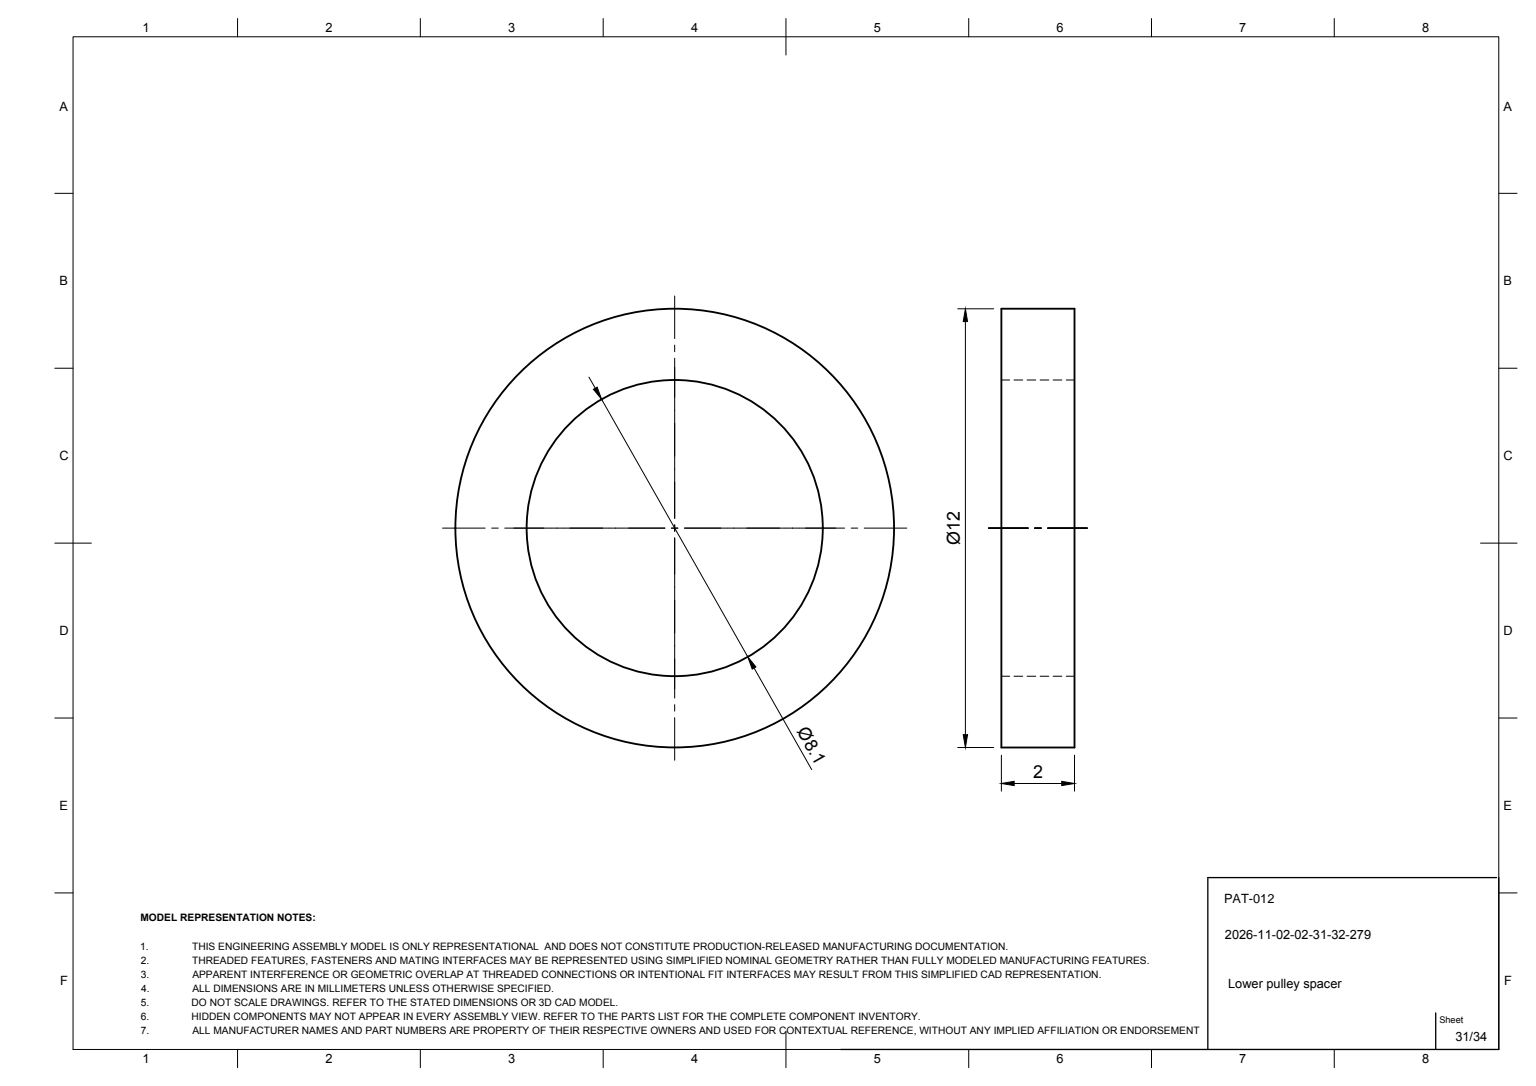
ISO-10303-21;
HEADER;
/* Generated by software containing ST-Developer
 * from STEP Tools, Inc. (www.steptools.com) 
 */

FILE_DESCRIPTION(
/* description */ ('Belt tensioner idler arm'),
/* implementation_level */ '2;1');

FILE_NAME(
/* name */ 'Lower pulley spacer.step',
/* time_stamp */ '2026-10-28T03:22:15-07:00',
/* author */ (''),
/* organization */ (''),
/* preprocessor_version */ 'ST-DEVELOPER v20.2',
/* originating_system */ 'Autodesk Translation Framework v15.17.0.0',
/* authorisation */ '');

FILE_SCHEMA (('AUTOMOTIVE_DESIGN { 1 0 10303 214 3 1 1 }'));
ENDSEC;

DATA;
#10=MECHANICAL_DESIGN_GEOMETRIC_PRESENTATION_REPRESENTATION('',(#481),#12779);
#405=SHAPE_REPRESENTATION_RELATIONSHIP('SRR','None',#12954,#439);
#439=ADVANCED_BREP_SHAPE_REPRESENTATION('',(#520),#12771);
#481=STYLED_ITEM('',(#13177),#520);
#520=MANIFOLD_SOLID_BREP('Body1',#6218);
#644=FACE_BOUND('',#1593,.T.);
#645=FACE_BOUND('',#1595,.T.);
#802=PLANE('',#7188);
#803=PLANE('',#7189);
#1106=FACE_OUTER_BOUND('',#1590,.T.);
#1107=FACE_OUTER_BOUND('',#1591,.T.);
#1108=FACE_OUTER_BOUND('',#1592,.T.);
#1109=FACE_OUTER_BOUND('',#1594,.T.);
#1590=EDGE_LOOP('',(#5188,#5189,#5190,#5191));
#1591=EDGE_LOOP('',(#5192,#5193,#5194,#5195));
#1592=EDGE_LOOP('',(#5196));
#1593=EDGE_LOOP('',(#5197));
#1594=EDGE_LOOP('',(#5198));
#1595=EDGE_LOOP('',(#5199));
#1955=LINE('',#11892,#2304);
#1956=LINE('',#11898,#2305);
#2304=VECTOR('',#8845,0.404999999999999);
#2305=VECTOR('',#8852,0.6);
#2655=CIRCLE('',#7183,0.404999999999999);
#2656=CIRCLE('',#7184,0.404999999999999);
#2657=CIRCLE('',#7186,0.6);
#2658=CIRCLE('',#7187,0.6);
#3138=VERTEX_POINT('',#11889);
#3139=VERTEX_POINT('',#11891);
#3140=VERTEX_POINT('',#11895);
#3141=VERTEX_POINT('',#11897);
#3849=EDGE_CURVE('',#3138,#3138,#2655,.T.);
#3850=EDGE_CURVE('',#3138,#3139,#1955,.T.);
#3851=EDGE_CURVE('',#3139,#3139,#2656,.T.);
#3852=EDGE_CURVE('',#3140,#3140,#2657,.T.);
#3853=EDGE_CURVE('',#3140,#3141,#1956,.T.);
#3854=EDGE_CURVE('',#3141,#3141,#2658,.T.);
#5188=ORIENTED_EDGE('',*,*,#3849,.F.);
#5189=ORIENTED_EDGE('',*,*,#3850,.T.);
#5190=ORIENTED_EDGE('',*,*,#3851,.T.);
#5191=ORIENTED_EDGE('',*,*,#3850,.F.);
#5192=ORIENTED_EDGE('',*,*,#3852,.F.);
#5193=ORIENTED_EDGE('',*,*,#3853,.T.);
#5194=ORIENTED_EDGE('',*,*,#3854,.T.);
#5195=ORIENTED_EDGE('',*,*,#3853,.F.);
#5196=ORIENTED_EDGE('',*,*,#3852,.T.);
#5197=ORIENTED_EDGE('',*,*,#3849,.T.);
#5198=ORIENTED_EDGE('',*,*,#3854,.F.);
#5199=ORIENTED_EDGE('',*,*,#3851,.F.);
#5755=CYLINDRICAL_SURFACE('',#7182,0.404999999999999);
#5756=CYLINDRICAL_SURFACE('',#7185,0.6);
#6083=ADVANCED_FACE('',(#1106),#5755,.F.);
#6084=ADVANCED_FACE('',(#1107),#5756,.T.);
#6085=ADVANCED_FACE('',(#1108,#644),#802,.T.);
#6086=ADVANCED_FACE('',(#1109,#645),#803,.F.);
#6218=CLOSED_SHELL('',(#6083,#6084,#6085,#6086));
#7181=AXIS2_PLACEMENT_3D('',#11887,#8839,#8840);
#7182=AXIS2_PLACEMENT_3D('',#11888,#8841,#8842);
#7183=AXIS2_PLACEMENT_3D('',#11890,#8843,#8844);
#7184=AXIS2_PLACEMENT_3D('',#11893,#8846,#8847);
#7185=AXIS2_PLACEMENT_3D('',#11894,#8848,#8849);
#7186=AXIS2_PLACEMENT_3D('',#11896,#8850,#8851);
#7187=AXIS2_PLACEMENT_3D('',#11899,#8853,#8854);
#7188=AXIS2_PLACEMENT_3D('',#11900,#8855,#8856);
#7189=AXIS2_PLACEMENT_3D('',#11901,#8857,#8858);
#8839=DIRECTION('axis',(0.,0.,1.));
#8840=DIRECTION('refdir',(1.,0.,0.));
#8841=DIRECTION('center_axis',(0.,0.,1.));
#8842=DIRECTION('ref_axis',(1.,0.,0.));
#8843=DIRECTION('center_axis',(0.,0.,-1.));
#8844=DIRECTION('ref_axis',(1.,0.,0.));
#8845=DIRECTION('',(0.,0.,-1.));
#8846=DIRECTION('center_axis',(0.,0.,-1.));
#8847=DIRECTION('ref_axis',(1.,0.,0.));
#8848=DIRECTION('center_axis',(0.,0.,1.));
#8849=DIRECTION('ref_axis',(1.,0.,0.));
#8850=DIRECTION('center_axis',(0.,0.,1.));
#8851=DIRECTION('ref_axis',(1.,0.,0.));
#8852=DIRECTION('',(0.,0.,-1.));
#8853=DIRECTION('center_axis',(0.,0.,1.));
#8854=DIRECTION('ref_axis',(1.,0.,0.));
#8855=DIRECTION('center_axis',(0.,0.,1.));
#8856=DIRECTION('ref_axis',(1.,0.,0.));
#8857=DIRECTION('center_axis',(0.,0.,1.));
#8858=DIRECTION('ref_axis',(1.,0.,0.));
#11887=CARTESIAN_POINT('',(0.,0.,0.));
#11888=CARTESIAN_POINT('Origin',(9.,0.,7.));
#11889=CARTESIAN_POINT('',(8.595,-4.95981953654677E-17,7.2));
#11890=CARTESIAN_POINT('Origin',(9.,0.,7.2));
#11891=CARTESIAN_POINT('',(8.595,-4.95981953654677E-17,7.));
#11892=CARTESIAN_POINT('',(8.595,-4.95981953654677E-17,7.));
#11893=CARTESIAN_POINT('Origin',(9.,0.,7.));
#11894=CARTESIAN_POINT('Origin',(9.,0.,7.));
#11895=CARTESIAN_POINT('',(8.4,-7.34788079488412E-17,7.2));
#11896=CARTESIAN_POINT('Origin',(9.,0.,7.2));
#11897=CARTESIAN_POINT('',(8.4,-7.34788079488412E-17,7.));
#11898=CARTESIAN_POINT('',(8.4,-7.34788079488412E-17,7.));
#11899=CARTESIAN_POINT('Origin',(9.,0.,7.));
#11900=CARTESIAN_POINT('Origin',(9.,0.,7.2));
#11901=CARTESIAN_POINT('Origin',(9.,0.,7.));
#12731=UNCERTAINTY_MEASURE_WITH_UNIT(LENGTH_MEASURE(0.001),#12780,
'DISTANCE_ACCURACY_VALUE',
'Maximum model space distance between geometric entities at asserted c
onnectivities');
#12739=UNCERTAINTY_MEASURE_WITH_UNIT(LENGTH_MEASURE(0.001),#12780,
'DISTANCE_ACCURACY_VALUE',
'Maximum model space distance between geometric entities at asserted c
onnectivities');
#12771=(
GEOMETRIC_REPRESENTATION_CONTEXT(3)
GLOBAL_UNCERTAINTY_ASSIGNED_CONTEXT((#12731))
GLOBAL_UNIT_ASSIGNED_CONTEXT((#12780,#12782,#12783))
REPRESENTATION_CONTEXT('','3D')
);
#12779=(
GEOMETRIC_REPRESENTATION_CONTEXT(3)
GLOBAL_UNCERTAINTY_ASSIGNED_CONTEXT((#12739))
GLOBAL_UNIT_ASSIGNED_CONTEXT((#12780,#12782,#12783))
REPRESENTATION_CONTEXT('','3D')
);
#12780=(
LENGTH_UNIT()
NAMED_UNIT(*)
SI_UNIT(.CENTI.,.METRE.)
);
#12782=(
NAMED_UNIT(*)
PLANE_ANGLE_UNIT()
SI_UNIT($,.RADIAN.)
);
#12783=(
NAMED_UNIT(*)
SI_UNIT($,.STERADIAN.)
SOLID_ANGLE_UNIT()
);
#12815=SHAPE_DEFINITION_REPRESENTATION(#12883,#12954);
#12883=PRODUCT_DEFINITION_SHAPE('',$,#12994);
#12954=SHAPE_REPRESENTATION('',(#7181),#12771);
#12962=PRODUCT_DEFINITION_CONTEXT('part definition',#13081,'design');
#12994=PRODUCT_DEFINITION('Lower pulley spacer','Lower pulley spacer',#13033,
#12962);
#13033=PRODUCT_DEFINITION_FORMATION('',$,#13114);
#13081=APPLICATION_CONTEXT(
'Core Data for Automotive Mechanical Design Process');
#13082=PRODUCT_CONTEXT('part definition',#13081,'mechanical');
#13114=PRODUCT('Lower pulley spacer','Lower pulley spacer',
'Lower pulley spacer',(#13082));
#13171=COLOUR_RGB('Sky Blue',0.24,0.69,0.87);
#13172=FILL_AREA_STYLE_COLOUR('',#13171);
#13173=FILL_AREA_STYLE('',(#13172));
#13174=SURFACE_STYLE_FILL_AREA(#13173);
#13175=SURFACE_SIDE_STYLE('',(#13174));
#13176=SURFACE_STYLE_USAGE(.BOTH.,#13175);
#13177=PRESENTATION_STYLE_ASSIGNMENT((#13176));
ENDSEC;
END-ISO-10303-21;
